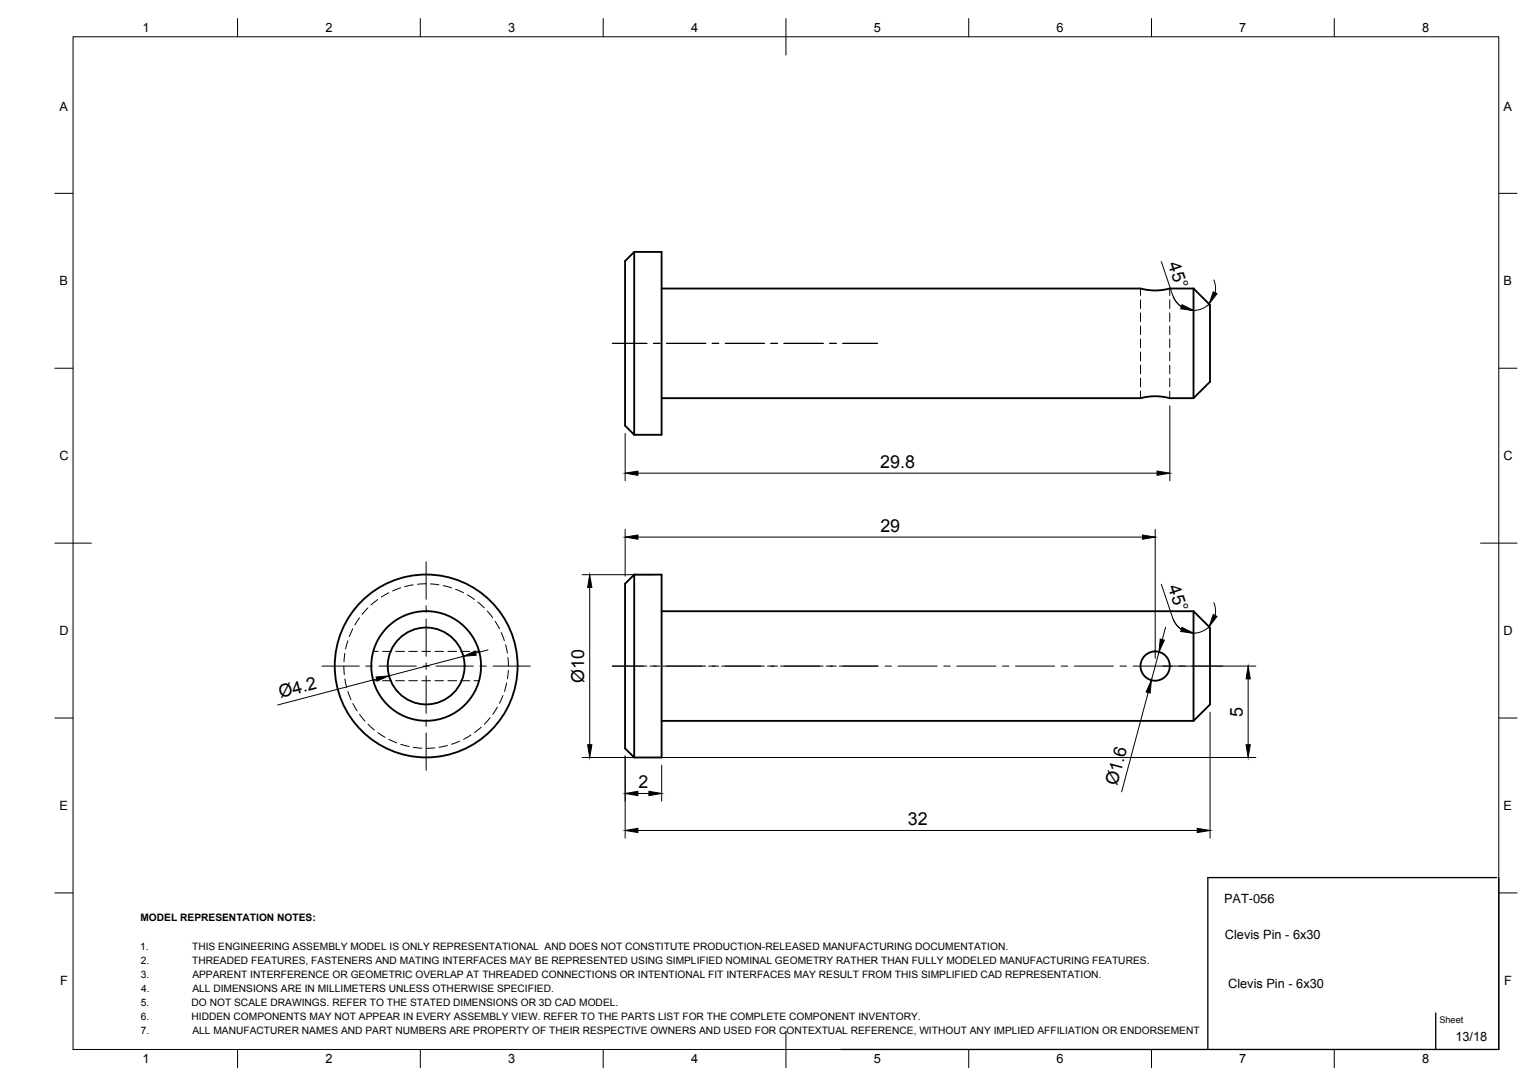
ISO-10303-21;
HEADER;
/* Generated by software containing ST-Developer
 * from STEP Tools, Inc. (www.steptools.com) 
 */

FILE_DESCRIPTION(
/* description */ ('Hook toggle clamp'),
/* implementation_level */ '2;1');

FILE_NAME(
/* name */ 'Clevis Pin - 6x30.step',
/* time_stamp */ '2026-10-27T21:56:56-07:00',
/* author */ (''),
/* organization */ (''),
/* preprocessor_version */ 'ST-DEVELOPER v20.2',
/* originating_system */ 'Autodesk Translation Framework v15.17.0.0',
/* authorisation */ '');

FILE_SCHEMA (('AUTOMOTIVE_DESIGN { 1 0 10303 214 3 1 1 }'));
ENDSEC;

DATA;
#10=MECHANICAL_DESIGN_GEOMETRIC_PRESENTATION_REPRESENTATION('',(#200),#5458);
#13=B_SPLINE_CURVE_WITH_KNOTS('',3,(#5084,#5085,#5086,#5087,#5088,#5089,
#5090,#5091,#5092,#5093),.UNSPECIFIED.,.F.,.F.,(4,2,2,2,4),(0.,0.0302963256060356,
0.0605926512120712,0.090883446720838,0.121174242229605),.UNSPECIFIED.);
#14=B_SPLINE_CURVE_WITH_KNOTS('',3,(#5096,#5097,#5098,#5099,#5100,#5101,
#5102,#5103,#5104,#5105,#5106,#5107,#5108,#5109,#5110,#5111,#5112,#5113,
#5114,#5115,#5116,#5117,#5118,#5119,#5120,#5121,#5122,#5123,#5124,#5125,
#5126,#5127,#5128,#5129),.UNSPECIFIED.,.T.,.F.,(4,2,2,2,2,2,2,2,2,2,2,2,
2,2,2,2,4),(0.,0.0302963256060358,0.0605926512120716,0.0908834467208383,
0.121174242229605,0.151465037738372,0.181755833247138,0.212052158853174,
0.24234848445921,0.272644810065246,0.302941135671282,0.333231931180048,
0.363522726688815,0.393813522197582,0.424104317706349,0.454400643312384,
0.48469696891842),.UNSPECIFIED.);
#15=B_SPLINE_CURVE_WITH_KNOTS('',3,(#5131,#5132,#5133,#5134,#5135,#5136,
#5137,#5138,#5139,#5140),.UNSPECIFIED.,.F.,.F.,(4,2,2,2,4),(0.363522726688815,
0.393813522197581,0.424104317706348,0.454400643312384,0.48469696891842),
 .UNSPECIFIED.);
#16=B_SPLINE_CURVE_WITH_KNOTS('',3,(#5141,#5142,#5143,#5144,#5145,#5146,
#5147,#5148,#5149,#5150,#5151,#5152,#5153,#5154,#5155,#5156,#5157,#5158),
 .UNSPECIFIED.,.F.,.F.,(4,2,2,2,2,2,2,2,4),(0.121174242229605,0.151465037738371,
0.181755833247138,0.212052158853174,0.24234848445921,0.272644810065246,
0.302941135671281,0.333231931180048,0.363522726688815),.UNSPECIFIED.);
#151=CONICAL_SURFACE('',#3416,0.475,0.785398163397448);
#152=CONICAL_SURFACE('',#3424,0.255,0.785398163397449);
#166=SHAPE_REPRESENTATION_RELATIONSHIP('SRR','None',#5550,#183);
#183=ADVANCED_BREP_SHAPE_REPRESENTATION('',(#216),#5452);
#200=STYLED_ITEM('',(#5717),#216);
#216=MANIFOLD_SOLID_BREP('Body1',#2982);
#269=FACE_BOUND('',#754,.T.);
#270=FACE_BOUND('',#756,.T.);
#373=PLANE('',#3414);
#374=PLANE('',#3420);
#375=PLANE('',#3426);
#529=FACE_OUTER_BOUND('',#749,.T.);
#530=FACE_OUTER_BOUND('',#750,.T.);
#531=FACE_OUTER_BOUND('',#751,.T.);
#532=FACE_OUTER_BOUND('',#752,.T.);
#533=FACE_OUTER_BOUND('',#753,.T.);
#534=FACE_OUTER_BOUND('',#755,.T.);
#535=FACE_OUTER_BOUND('',#757,.T.);
#536=FACE_OUTER_BOUND('',#758,.T.);
#749=EDGE_LOOP('',(#2601,#2602,#2603,#2604,#2605,#2606));
#750=EDGE_LOOP('',(#2607));
#751=EDGE_LOOP('',(#2608,#2609,#2610,#2611));
#752=EDGE_LOOP('',(#2612,#2613,#2614,#2615));
#753=EDGE_LOOP('',(#2616));
#754=EDGE_LOOP('',(#2617));
#755=EDGE_LOOP('',(#2618,#2619,#2620,#2621,#2622,#2623,#2624,#2625,#2626));
#756=EDGE_LOOP('',(#2627));
#757=EDGE_LOOP('',(#2628,#2629,#2630,#2631));
#758=EDGE_LOOP('',(#2632));
#1006=LINE('',#5095,#1243);
#1007=LINE('',#5165,#1244);
#1008=LINE('',#5169,#1245);
#1009=LINE('',#5176,#1246);
#1010=LINE('',#5177,#1247);
#1011=LINE('',#5181,#1248);
#1243=VECTOR('',#4198,0.08);
#1244=VECTOR('',#4207,0.475);
#1245=VECTOR('',#4212,0.5);
#1246=VECTOR('',#4221,0.3);
#1247=VECTOR('',#4222,0.3);
#1248=VECTOR('',#4227,0.255);
#1352=CIRCLE('',#3415,0.45);
#1353=CIRCLE('',#3417,0.5);
#1354=CIRCLE('',#3419,0.5);
#1355=CIRCLE('',#3421,0.3);
#1356=CIRCLE('',#3423,0.3);
#1357=CIRCLE('',#3425,0.21);
#1579=VERTEX_POINT('',#5082);
#1580=VERTEX_POINT('',#5083);
#1581=VERTEX_POINT('',#5094);
#1582=VERTEX_POINT('',#5130);
#1583=VERTEX_POINT('',#5160);
#1584=VERTEX_POINT('',#5163);
#1585=VERTEX_POINT('',#5167);
#1586=VERTEX_POINT('',#5171);
#1587=VERTEX_POINT('',#5174);
#1588=VERTEX_POINT('',#5179);
#1927=EDGE_CURVE('',#1579,#1580,#13,.T.);
#1928=EDGE_CURVE('',#1579,#1581,#1006,.T.);
#1929=EDGE_CURVE('',#1581,#1581,#14,.T.);
#1930=EDGE_CURVE('',#1582,#1579,#15,.T.);
#1931=EDGE_CURVE('',#1580,#1582,#16,.T.);
#1932=EDGE_CURVE('',#1583,#1583,#1352,.T.);
#1933=EDGE_CURVE('',#1584,#1584,#1353,.T.);
#1934=EDGE_CURVE('',#1584,#1583,#1007,.T.);
#1935=EDGE_CURVE('',#1585,#1585,#1354,.T.);
#1936=EDGE_CURVE('',#1585,#1584,#1008,.T.);
#1937=EDGE_CURVE('',#1586,#1586,#1355,.T.);
#1938=EDGE_CURVE('',#1587,#1587,#1356,.T.);
#1939=EDGE_CURVE('',#1587,#1580,#1009,.T.);
#1940=EDGE_CURVE('',#1582,#1586,#1010,.T.);
#1941=EDGE_CURVE('',#1588,#1588,#1357,.T.);
#1942=EDGE_CURVE('',#1588,#1587,#1011,.T.);
#2601=ORIENTED_EDGE('',*,*,#1927,.F.);
#2602=ORIENTED_EDGE('',*,*,#1928,.T.);
#2603=ORIENTED_EDGE('',*,*,#1929,.F.);
#2604=ORIENTED_EDGE('',*,*,#1928,.F.);
#2605=ORIENTED_EDGE('',*,*,#1930,.F.);
#2606=ORIENTED_EDGE('',*,*,#1931,.F.);
#2607=ORIENTED_EDGE('',*,*,#1932,.F.);
#2608=ORIENTED_EDGE('',*,*,#1933,.F.);
#2609=ORIENTED_EDGE('',*,*,#1934,.T.);
#2610=ORIENTED_EDGE('',*,*,#1932,.T.);
#2611=ORIENTED_EDGE('',*,*,#1934,.F.);
#2612=ORIENTED_EDGE('',*,*,#1935,.F.);
#2613=ORIENTED_EDGE('',*,*,#1936,.T.);
#2614=ORIENTED_EDGE('',*,*,#1933,.T.);
#2615=ORIENTED_EDGE('',*,*,#1936,.F.);
#2616=ORIENTED_EDGE('',*,*,#1935,.T.);
#2617=ORIENTED_EDGE('',*,*,#1937,.F.);
#2618=ORIENTED_EDGE('',*,*,#1938,.F.);
#2619=ORIENTED_EDGE('',*,*,#1939,.T.);
#2620=ORIENTED_EDGE('',*,*,#1931,.T.);
#2621=ORIENTED_EDGE('',*,*,#1940,.T.);
#2622=ORIENTED_EDGE('',*,*,#1937,.T.);
#2623=ORIENTED_EDGE('',*,*,#1940,.F.);
#2624=ORIENTED_EDGE('',*,*,#1930,.T.);
#2625=ORIENTED_EDGE('',*,*,#1927,.T.);
#2626=ORIENTED_EDGE('',*,*,#1939,.F.);
#2627=ORIENTED_EDGE('',*,*,#1929,.T.);
#2628=ORIENTED_EDGE('',*,*,#1941,.F.);
#2629=ORIENTED_EDGE('',*,*,#1942,.T.);
#2630=ORIENTED_EDGE('',*,*,#1938,.T.);
#2631=ORIENTED_EDGE('',*,*,#1942,.F.);
#2632=ORIENTED_EDGE('',*,*,#1941,.T.);
#2786=CYLINDRICAL_SURFACE('',#3413,0.08);
#2787=CYLINDRICAL_SURFACE('',#3418,0.5);
#2788=CYLINDRICAL_SURFACE('',#3422,0.3);
#2933=ADVANCED_FACE('',(#529),#2786,.F.);
#2934=ADVANCED_FACE('',(#530),#373,.T.);
#2935=ADVANCED_FACE('',(#531),#151,.T.);
#2936=ADVANCED_FACE('',(#532),#2787,.T.);
#2937=ADVANCED_FACE('',(#533,#269),#374,.T.);
#2938=ADVANCED_FACE('',(#534,#270),#2788,.T.);
#2939=ADVANCED_FACE('',(#535),#152,.T.);
#2940=ADVANCED_FACE('',(#536),#375,.T.);
#2982=CLOSED_SHELL('',(#2933,#2934,#2935,#2936,#2937,#2938,#2939,#2940));
#3412=AXIS2_PLACEMENT_3D('',#5080,#4194,#4195);
#3413=AXIS2_PLACEMENT_3D('',#5081,#4196,#4197);
#3414=AXIS2_PLACEMENT_3D('',#5159,#4199,#4200);
#3415=AXIS2_PLACEMENT_3D('',#5161,#4201,#4202);
#3416=AXIS2_PLACEMENT_3D('',#5162,#4203,#4204);
#3417=AXIS2_PLACEMENT_3D('',#5164,#4205,#4206);
#3418=AXIS2_PLACEMENT_3D('',#5166,#4208,#4209);
#3419=AXIS2_PLACEMENT_3D('',#5168,#4210,#4211);
#3420=AXIS2_PLACEMENT_3D('',#5170,#4213,#4214);
#3421=AXIS2_PLACEMENT_3D('',#5172,#4215,#4216);
#3422=AXIS2_PLACEMENT_3D('',#5173,#4217,#4218);
#3423=AXIS2_PLACEMENT_3D('',#5175,#4219,#4220);
#3424=AXIS2_PLACEMENT_3D('',#5178,#4223,#4224);
#3425=AXIS2_PLACEMENT_3D('',#5180,#4225,#4226);
#3426=AXIS2_PLACEMENT_3D('',#5182,#4228,#4229);
#4194=DIRECTION('axis',(0.,0.,1.));
#4195=DIRECTION('refdir',(1.,0.,0.));
#4196=DIRECTION('center_axis',(1.,0.,0.));
#4197=DIRECTION('ref_axis',(0.,0.,-1.));
#4198=DIRECTION('',(1.,0.,0.));
#4199=DIRECTION('center_axis',(0.,1.,0.));
#4200=DIRECTION('ref_axis',(0.,0.,1.));
#4201=DIRECTION('center_axis',(0.,-1.,0.));
#4202=DIRECTION('ref_axis',(1.,0.,0.));
#4203=DIRECTION('center_axis',(0.,-1.,0.));
#4204=DIRECTION('ref_axis',(1.,0.,0.));
#4205=DIRECTION('center_axis',(0.,-1.,0.));
#4206=DIRECTION('ref_axis',(1.,0.,0.));
#4207=DIRECTION('',(0.707106781186547,0.707106781186548,8.65956056235493E-17));
#4208=DIRECTION('center_axis',(0.,-1.,0.));
#4209=DIRECTION('ref_axis',(1.,0.,0.));
#4210=DIRECTION('center_axis',(0.,-1.,0.));
#4211=DIRECTION('ref_axis',(1.,0.,0.));
#4212=DIRECTION('',(0.,1.,0.));
#4213=DIRECTION('center_axis',(0.,-1.,0.));
#4214=DIRECTION('ref_axis',(0.,0.,-1.));
#4215=DIRECTION('center_axis',(0.,-1.,0.));
#4216=DIRECTION('ref_axis',(1.,0.,0.));
#4217=DIRECTION('center_axis',(0.,-1.,0.));
#4218=DIRECTION('ref_axis',(1.,0.,0.));
#4219=DIRECTION('center_axis',(0.,-1.,0.));
#4220=DIRECTION('ref_axis',(1.,0.,0.));
#4221=DIRECTION('',(0.,1.,0.));
#4222=DIRECTION('',(0.,1.,0.));
#4223=DIRECTION('center_axis',(0.,1.,0.));
#4224=DIRECTION('ref_axis',(1.,0.,0.));
#4225=DIRECTION('center_axis',(0.,-1.,0.));
#4226=DIRECTION('ref_axis',(1.,0.,0.));
#4227=DIRECTION('',(-0.707106781186548,0.707106781186547,-8.65956056235494E-17));
#4228=DIRECTION('center_axis',(0.,-1.,0.));
#4229=DIRECTION('ref_axis',(0.,0.,-1.));
#5080=CARTESIAN_POINT('',(0.,0.,0.));
#5081=CARTESIAN_POINT('Origin',(0.,-2.7,0.));
#5082=CARTESIAN_POINT('',(-0.289136645896019,-2.7,0.08));
#5083=CARTESIAN_POINT('',(-0.3,-2.78,-2.27065106771523E-17));
#5084=CARTESIAN_POINT('Ctrl Pts',(-0.289136645896019,-2.7,0.08));
#5085=CARTESIAN_POINT('Ctrl Pts',(-0.289136645896019,-2.71009877520201,
0.08));
#5086=CARTESIAN_POINT('Ctrl Pts',(-0.289720927595908,-2.72083518625944,
0.0779717130936404));
#5087=CARTESIAN_POINT('Ctrl Pts',(-0.291799203044223,-2.74052980652726,
0.0697927537456149));
#5088=CARTESIAN_POINT('Ctrl Pts',(-0.293259762986909,-2.74949254880105,
0.0636445361887959));
#5089=CARTESIAN_POINT('Ctrl Pts',(-0.295976783522942,-2.76364324458222,
0.0494938404076284));
#5090=CARTESIAN_POINT('Ctrl Pts',(-0.297414335384467,-2.76979246713824,
0.0405305642602551));
#5091=CARTESIAN_POINT('Ctrl Pts',(-0.299439403644655,-2.77797216257078,
0.0208340363410407));
#5092=CARTESIAN_POINT('Ctrl Pts',(-0.3,-2.78,0.0100969318362556));
#5093=CARTESIAN_POINT('Ctrl Pts',(-0.3,-2.78,5.20417042793042E-18));
#5094=CARTESIAN_POINT('',(0.289136645896019,-2.7,0.08));
#5095=CARTESIAN_POINT('',(0.,-2.7,0.08));
#5096=CARTESIAN_POINT('Ctrl Pts',(0.289136645896019,-2.7,0.08));
#5097=CARTESIAN_POINT('Ctrl Pts',(0.289136645896019,-2.68990122479799,0.08));
#5098=CARTESIAN_POINT('Ctrl Pts',(0.289720927595908,-2.67916481374056,0.0779717130936404));
#5099=CARTESIAN_POINT('Ctrl Pts',(0.291799203044223,-2.65947019347274,0.0697927537456147));
#5100=CARTESIAN_POINT('Ctrl Pts',(0.293259762986909,-2.65050745119895,0.0636445361887959));
#5101=CARTESIAN_POINT('Ctrl Pts',(0.295976783522942,-2.63635675541778,0.0494938404076283));
#5102=CARTESIAN_POINT('Ctrl Pts',(0.297414335384467,-2.63020753286176,0.0405305642602551));
#5103=CARTESIAN_POINT('Ctrl Pts',(0.299439403644655,-2.62202783742922,0.0208340363410406));
#5104=CARTESIAN_POINT('Ctrl Pts',(0.3,-2.62,0.0100969318362555));
#5105=CARTESIAN_POINT('Ctrl Pts',(0.3,-2.62,-0.0100969318362556));
#5106=CARTESIAN_POINT('Ctrl Pts',(0.299439403644655,-2.62202783742922,-0.0208340363410406));
#5107=CARTESIAN_POINT('Ctrl Pts',(0.297414335384467,-2.63020753286176,-0.0405305642602551));
#5108=CARTESIAN_POINT('Ctrl Pts',(0.295976783522942,-2.63635675541778,-0.0494938404076283));
#5109=CARTESIAN_POINT('Ctrl Pts',(0.293259762986909,-2.65050745119895,-0.0636445361887959));
#5110=CARTESIAN_POINT('Ctrl Pts',(0.291799203044223,-2.65947019347274,-0.0697927537456147));
#5111=CARTESIAN_POINT('Ctrl Pts',(0.289720927595908,-2.67916481374056,-0.0779717130936403));
#5112=CARTESIAN_POINT('Ctrl Pts',(0.289136645896019,-2.68990122479799,-0.08));
#5113=CARTESIAN_POINT('Ctrl Pts',(0.289136645896019,-2.71009877520201,-0.08));
#5114=CARTESIAN_POINT('Ctrl Pts',(0.289720927595908,-2.72083518625944,-0.0779717130936404));
#5115=CARTESIAN_POINT('Ctrl Pts',(0.291799203044223,-2.74052980652726,-0.0697927537456147));
#5116=CARTESIAN_POINT('Ctrl Pts',(0.293259762986909,-2.74949254880105,-0.0636445361887959));
#5117=CARTESIAN_POINT('Ctrl Pts',(0.295976783522942,-2.76364324458222,-0.0494938404076283));
#5118=CARTESIAN_POINT('Ctrl Pts',(0.297414335384467,-2.76979246713824,-0.0405305642602551));
#5119=CARTESIAN_POINT('Ctrl Pts',(0.299439403644655,-2.77797216257078,-0.0208340363410406));
#5120=CARTESIAN_POINT('Ctrl Pts',(0.3,-2.78,-0.0100969318362555));
#5121=CARTESIAN_POINT('Ctrl Pts',(0.3,-2.78,0.0100969318362556));
#5122=CARTESIAN_POINT('Ctrl Pts',(0.299439403644655,-2.77797216257078,0.0208340363410407));
#5123=CARTESIAN_POINT('Ctrl Pts',(0.297414335384467,-2.76979246713824,0.0405305642602551));
#5124=CARTESIAN_POINT('Ctrl Pts',(0.295976783522942,-2.76364324458222,0.0494938404076284));
#5125=CARTESIAN_POINT('Ctrl Pts',(0.293259762986909,-2.74949254880105,0.0636445361887959));
#5126=CARTESIAN_POINT('Ctrl Pts',(0.291799203044223,-2.74052980652726,0.0697927537456149));
#5127=CARTESIAN_POINT('Ctrl Pts',(0.289720927595908,-2.72083518625944,0.0779717130936404));
#5128=CARTESIAN_POINT('Ctrl Pts',(0.289136645896019,-2.71009877520201,0.08));
#5129=CARTESIAN_POINT('Ctrl Pts',(0.289136645896019,-2.7,0.08));
#5130=CARTESIAN_POINT('',(-0.3,-2.62,-3.65842984849668E-17));
#5131=CARTESIAN_POINT('Ctrl Pts',(-0.3,-2.62,-3.81639164714898E-17));
#5132=CARTESIAN_POINT('Ctrl Pts',(-0.3,-2.62,0.0100969318362555));
#5133=CARTESIAN_POINT('Ctrl Pts',(-0.299439403644655,-2.62202783742922,
0.0208340363410406));
#5134=CARTESIAN_POINT('Ctrl Pts',(-0.297414335384467,-2.63020753286176,
0.040530564260255));
#5135=CARTESIAN_POINT('Ctrl Pts',(-0.295976783522942,-2.63635675541778,
0.0494938404076283));
#5136=CARTESIAN_POINT('Ctrl Pts',(-0.293259762986909,-2.65050745119895,
0.0636445361887959));
#5137=CARTESIAN_POINT('Ctrl Pts',(-0.291799203044223,-2.65947019347274,
0.0697927537456147));
#5138=CARTESIAN_POINT('Ctrl Pts',(-0.289720927595908,-2.67916481374056,
0.0779717130936404));
#5139=CARTESIAN_POINT('Ctrl Pts',(-0.289136645896019,-2.68990122479799,
0.08));
#5140=CARTESIAN_POINT('Ctrl Pts',(-0.289136645896019,-2.7,0.08));
#5141=CARTESIAN_POINT('Ctrl Pts',(-0.3,-2.78,-6.93889390390723E-18));
#5142=CARTESIAN_POINT('Ctrl Pts',(-0.3,-2.78,-0.0100969318362556));
#5143=CARTESIAN_POINT('Ctrl Pts',(-0.299439403644655,-2.77797216257078,
-0.0208340363410406));
#5144=CARTESIAN_POINT('Ctrl Pts',(-0.297414335384467,-2.76979246713824,
-0.0405305642602551));
#5145=CARTESIAN_POINT('Ctrl Pts',(-0.295976783522942,-2.76364324458222,
-0.0494938404076283));
#5146=CARTESIAN_POINT('Ctrl Pts',(-0.293259762986909,-2.74949254880105,
-0.0636445361887959));
#5147=CARTESIAN_POINT('Ctrl Pts',(-0.291799203044223,-2.74052980652726,
-0.0697927537456147));
#5148=CARTESIAN_POINT('Ctrl Pts',(-0.289720927595908,-2.72083518625944,
-0.0779717130936403));
#5149=CARTESIAN_POINT('Ctrl Pts',(-0.289136645896019,-2.71009877520201,
-0.08));
#5150=CARTESIAN_POINT('Ctrl Pts',(-0.289136645896019,-2.68990122479799,
-0.08));
#5151=CARTESIAN_POINT('Ctrl Pts',(-0.289720927595908,-2.67916481374056,
-0.0779717130936403));
#5152=CARTESIAN_POINT('Ctrl Pts',(-0.291799203044223,-2.65947019347274,
-0.0697927537456147));
#5153=CARTESIAN_POINT('Ctrl Pts',(-0.293259762986909,-2.65050745119895,
-0.0636445361887959));
#5154=CARTESIAN_POINT('Ctrl Pts',(-0.295976783522942,-2.63635675541778,
-0.0494938404076283));
#5155=CARTESIAN_POINT('Ctrl Pts',(-0.297414335384467,-2.63020753286176,
-0.0405305642602551));
#5156=CARTESIAN_POINT('Ctrl Pts',(-0.299439403644655,-2.62202783742922,
-0.0208340363410406));
#5157=CARTESIAN_POINT('Ctrl Pts',(-0.3,-2.62,-0.0100969318362556));
#5158=CARTESIAN_POINT('Ctrl Pts',(-0.3,-2.62,-1.56125112837913E-17));
#5159=CARTESIAN_POINT('Origin',(0.45,0.2,0.));
#5160=CARTESIAN_POINT('',(-0.45,0.2,-5.51091059616309E-17));
#5161=CARTESIAN_POINT('Origin',(0.,0.2,0.));
#5162=CARTESIAN_POINT('Origin',(0.,0.175,0.));
#5163=CARTESIAN_POINT('',(-0.5,0.15,-6.12323399573676E-17));
#5164=CARTESIAN_POINT('Origin',(0.,0.15,0.));
#5165=CARTESIAN_POINT('',(-0.475,0.175,-5.81707229594993E-17));
#5166=CARTESIAN_POINT('Origin',(0.,0.0750000000000002,0.));
#5167=CARTESIAN_POINT('',(-0.5,0.,-6.12323399573677E-17));
#5168=CARTESIAN_POINT('Origin',(0.,0.,0.));
#5169=CARTESIAN_POINT('',(-0.5,0.0750000000000002,-6.12323399573677E-17));
#5170=CARTESIAN_POINT('Origin',(0.3,0.,0.));
#5171=CARTESIAN_POINT('',(-0.3,0.,-3.67394039744206E-17));
#5172=CARTESIAN_POINT('Origin',(0.,0.,0.));
#5173=CARTESIAN_POINT('Origin',(0.,-1.455,0.));
#5174=CARTESIAN_POINT('',(-0.3,-2.91,-3.67394039744206E-17));
#5175=CARTESIAN_POINT('Origin',(0.,-2.91,0.));
#5176=CARTESIAN_POINT('',(-0.3,-1.455,-3.67394039744206E-17));
#5177=CARTESIAN_POINT('',(-0.3,-1.455,-3.67394039744206E-17));
#5178=CARTESIAN_POINT('Origin',(0.,-2.955,0.));
#5179=CARTESIAN_POINT('',(-0.21,-3.,-2.57175827820944E-17));
#5180=CARTESIAN_POINT('Origin',(0.,-3.,0.));
#5181=CARTESIAN_POINT('',(-0.255,-2.955,-3.12284933782575E-17));
#5182=CARTESIAN_POINT('Origin',(0.,-3.,0.));
#5429=UNCERTAINTY_MEASURE_WITH_UNIT(LENGTH_MEASURE(0.001),#5459,
'DISTANCE_ACCURACY_VALUE',
'Maximum model space distance between geometric entities at asserted c
onnectivities');
#5435=UNCERTAINTY_MEASURE_WITH_UNIT(LENGTH_MEASURE(0.001),#5459,
'DISTANCE_ACCURACY_VALUE',
'Maximum model space distance between geometric entities at asserted c
onnectivities');
#5452=(
GEOMETRIC_REPRESENTATION_CONTEXT(3)
GLOBAL_UNCERTAINTY_ASSIGNED_CONTEXT((#5429))
GLOBAL_UNIT_ASSIGNED_CONTEXT((#5459,#5461,#5462))
REPRESENTATION_CONTEXT('','3D')
);
#5458=(
GEOMETRIC_REPRESENTATION_CONTEXT(3)
GLOBAL_UNCERTAINTY_ASSIGNED_CONTEXT((#5435))
GLOBAL_UNIT_ASSIGNED_CONTEXT((#5459,#5461,#5462))
REPRESENTATION_CONTEXT('','3D')
);
#5459=(
LENGTH_UNIT()
NAMED_UNIT(*)
SI_UNIT(.CENTI.,.METRE.)
);
#5461=(
NAMED_UNIT(*)
PLANE_ANGLE_UNIT()
SI_UNIT($,.RADIAN.)
);
#5462=(
NAMED_UNIT(*)
SI_UNIT($,.STERADIAN.)
SOLID_ANGLE_UNIT()
);
#5479=SHAPE_DEFINITION_REPRESENTATION(#5502,#5550);
#5502=PRODUCT_DEFINITION_SHAPE('',$,#5573);
#5550=SHAPE_REPRESENTATION('',(#3412),#5452);
#5556=PRODUCT_DEFINITION_CONTEXT('part definition',#5624,'design');
#5573=PRODUCT_DEFINITION('Clevis Pin - 6x30','Clevis Pin - 6x30',#5595,
#5556);
#5595=PRODUCT_DEFINITION_FORMATION('',$,#5642);
#5624=APPLICATION_CONTEXT(
'Core Data for Automotive Mechanical Design Process');
#5625=PRODUCT_CONTEXT('part definition',#5624,'mechanical');
#5642=PRODUCT('Clevis Pin - 6x30','Clevis Pin - 6x30',
'Clevis Pin - 6x30',(#5625));
#5711=COLOUR_RGB('Grey',0.48,0.52,0.57);
#5712=FILL_AREA_STYLE_COLOUR('',#5711);
#5713=FILL_AREA_STYLE('',(#5712));
#5714=SURFACE_STYLE_FILL_AREA(#5713);
#5715=SURFACE_SIDE_STYLE('',(#5714));
#5716=SURFACE_STYLE_USAGE(.BOTH.,#5715);
#5717=PRESENTATION_STYLE_ASSIGNMENT((#5716));
ENDSEC;
END-ISO-10303-21;
